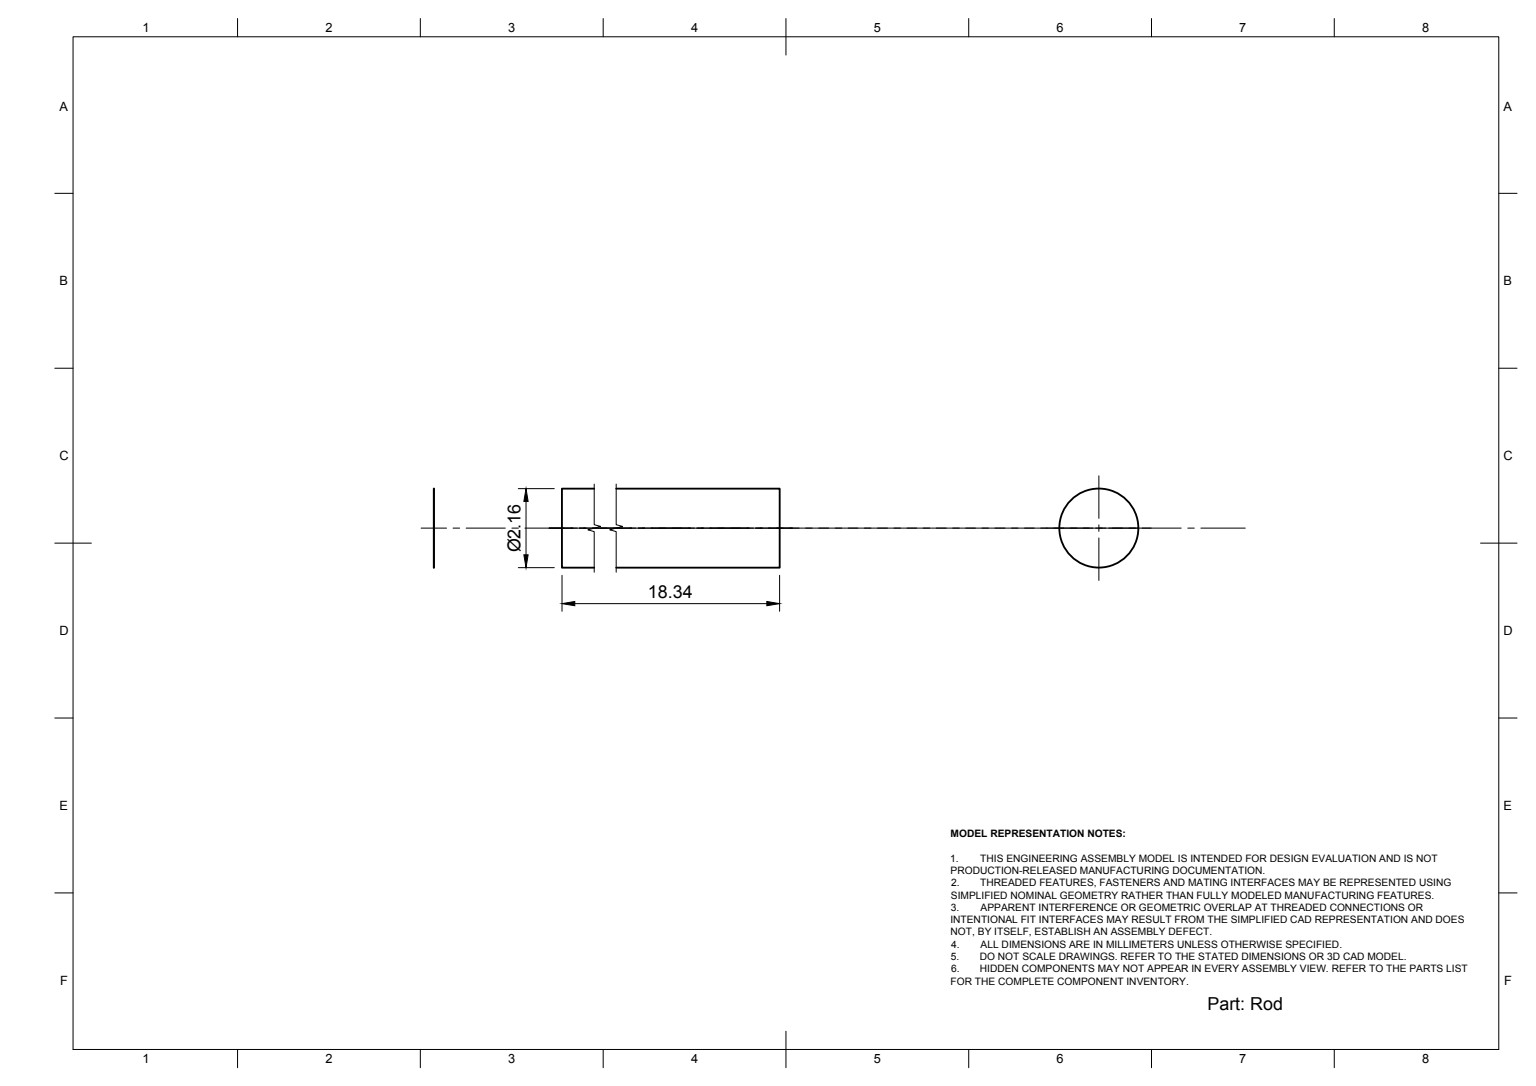
ISO-10303-21;
HEADER;
/* Generated by software containing ST-Developer
 * from STEP Tools, Inc. (www.steptools.com) 
 */

FILE_DESCRIPTION(
/* description */ (''),
/* implementation_level */ '2;1');

FILE_NAME(
/* name */ 'Rod.step',
/* time_stamp */ '2026-10-04T22:13:49-07:00',
/* author */ (''),
/* organization */ (''),
/* preprocessor_version */ 'ST-DEVELOPER v20.2',
/* originating_system */ 'Autodesk Translation Framework v15.15.0.0',
/* authorisation */ '');

FILE_SCHEMA (('AUTOMOTIVE_DESIGN { 1 0 10303 214 3 1 1 }'));
ENDSEC;

DATA;
#10=MECHANICAL_DESIGN_GEOMETRIC_PRESENTATION_REPRESENTATION('',(#365,#366),#40734);
#349=SHAPE_REPRESENTATION_RELATIONSHIP('SRR','None',#40770,#357);
#357=ADVANCED_BREP_SHAPE_REPRESENTATION('',(#374,#375),#40730);
#365=STYLED_ITEM('',(#40816),#374);
#366=STYLED_ITEM('',(#40816),#375);
#374=MANIFOLD_SOLID_BREP('Body1',#3170);
#375=MANIFOLD_SOLID_BREP('Body2',#3171);
#411=PLANE('',#3341);
#412=PLANE('',#3345);
#413=PLANE('',#3346);
#414=PLANE('',#3350);
#467=FACE_OUTER_BOUND('',#635,.T.);
#468=FACE_OUTER_BOUND('',#636,.T.);
#469=FACE_OUTER_BOUND('',#637,.T.);
#470=FACE_OUTER_BOUND('',#638,.T.);
#471=FACE_OUTER_BOUND('',#639,.T.);
#472=FACE_OUTER_BOUND('',#640,.T.);
#635=EDGE_LOOP('',(#2116));
#636=EDGE_LOOP('',(#2117,#2118,#2119,#2120));
#637=EDGE_LOOP('',(#2121));
#638=EDGE_LOOP('',(#2122));
#639=EDGE_LOOP('',(#2123,#2124,#2125,#2126));
#640=EDGE_LOOP('',(#2127));
#789=LINE('',#6473,#931);
#790=LINE('',#6481,#932);
#931=VECTOR('',#3674,1.08063175605657);
#932=VECTOR('',#3685,1.08063175605657);
#1074=CIRCLE('',#3342,1.08063175605657);
#1075=CIRCLE('',#3344,1.08063175605657);
#1076=CIRCLE('',#3347,1.08063175605657);
#1077=CIRCLE('',#3349,1.08063175605657);
#1159=VERTEX_POINT('',#6469);
#1160=VERTEX_POINT('',#6472);
#1161=VERTEX_POINT('',#6477);
#1162=VERTEX_POINT('',#6480);
#1534=EDGE_CURVE('',#1159,#1159,#1074,.T.);
#1535=EDGE_CURVE('',#1159,#1160,#789,.T.);
#1536=EDGE_CURVE('',#1160,#1160,#1075,.T.);
#1537=EDGE_CURVE('',#1161,#1161,#1076,.T.);
#1538=EDGE_CURVE('',#1161,#1162,#790,.T.);
#1539=EDGE_CURVE('',#1162,#1162,#1077,.T.);
#2116=ORIENTED_EDGE('',*,*,#1534,.F.);
#2117=ORIENTED_EDGE('',*,*,#1534,.T.);
#2118=ORIENTED_EDGE('',*,*,#1535,.T.);
#2119=ORIENTED_EDGE('',*,*,#1536,.T.);
#2120=ORIENTED_EDGE('',*,*,#1535,.F.);
#2121=ORIENTED_EDGE('',*,*,#1536,.F.);
#2122=ORIENTED_EDGE('',*,*,#1537,.T.);
#2123=ORIENTED_EDGE('',*,*,#1537,.F.);
#2124=ORIENTED_EDGE('',*,*,#1538,.T.);
#2125=ORIENTED_EDGE('',*,*,#1539,.T.);
#2126=ORIENTED_EDGE('',*,*,#1538,.F.);
#2127=ORIENTED_EDGE('',*,*,#1539,.F.);
#2908=CYLINDRICAL_SURFACE('',#3343,1.08063175605657);
#2909=CYLINDRICAL_SURFACE('',#3348,1.08063175605657);
#3046=ADVANCED_FACE('',(#467),#411,.F.);
#3047=ADVANCED_FACE('',(#468),#2908,.T.);
#3048=ADVANCED_FACE('',(#469),#412,.T.);
#3049=ADVANCED_FACE('',(#470),#413,.T.);
#3050=ADVANCED_FACE('',(#471),#2909,.T.);
#3051=ADVANCED_FACE('',(#472),#414,.T.);
#3170=CLOSED_SHELL('',(#3046,#3047,#3048));
#3171=CLOSED_SHELL('',(#3049,#3050,#3051));
#3340=AXIS2_PLACEMENT_3D('',#6467,#3666,#3667);
#3341=AXIS2_PLACEMENT_3D('',#6468,#3668,#3669);
#3342=AXIS2_PLACEMENT_3D('',#6470,#3670,#3671);
#3343=AXIS2_PLACEMENT_3D('',#6471,#3672,#3673);
#3344=AXIS2_PLACEMENT_3D('',#6474,#3675,#3676);
#3345=AXIS2_PLACEMENT_3D('',#6475,#3677,#3678);
#3346=AXIS2_PLACEMENT_3D('',#6476,#3679,#3680);
#3347=AXIS2_PLACEMENT_3D('',#6478,#3681,#3682);
#3348=AXIS2_PLACEMENT_3D('',#6479,#3683,#3684);
#3349=AXIS2_PLACEMENT_3D('',#6482,#3686,#3687);
#3350=AXIS2_PLACEMENT_3D('',#6483,#3688,#3689);
#3666=DIRECTION('axis',(0.,0.,1.));
#3667=DIRECTION('refdir',(1.,0.,0.));
#3668=DIRECTION('center_axis',(-1.,0.,0.));
#3669=DIRECTION('ref_axis',(0.,-1.,0.));
#3670=DIRECTION('center_axis',(-1.,0.,0.));
#3671=DIRECTION('ref_axis',(0.,0.,-1.));
#3672=DIRECTION('center_axis',(1.,0.,0.));
#3673=DIRECTION('ref_axis',(0.,0.,-1.));
#3674=DIRECTION('',(-1.,0.,0.));
#3675=DIRECTION('center_axis',(1.,0.,0.));
#3676=DIRECTION('ref_axis',(0.,0.,-1.));
#3677=DIRECTION('center_axis',(-1.,0.,0.));
#3678=DIRECTION('ref_axis',(0.,0.,1.));
#3679=DIRECTION('center_axis',(1.,0.,0.));
#3680=DIRECTION('ref_axis',(0.,0.,-1.));
#3681=DIRECTION('center_axis',(1.,0.,0.));
#3682=DIRECTION('ref_axis',(0.,0.,-1.));
#3683=DIRECTION('center_axis',(1.,0.,0.));
#3684=DIRECTION('ref_axis',(0.,0.,-1.));
#3685=DIRECTION('',(-1.,0.,0.));
#3686=DIRECTION('center_axis',(1.,0.,0.));
#3687=DIRECTION('ref_axis',(0.,0.,-1.));
#3688=DIRECTION('center_axis',(-1.,0.,0.));
#3689=DIRECTION('ref_axis',(0.,-1.,0.));
#6467=CARTESIAN_POINT('',(0.,0.,0.));
#6468=CARTESIAN_POINT('Origin',(85.6487002358236,0.,-8.18789480661053E-15));
#6469=CARTESIAN_POINT('',(85.6487002358236,-1.32339222111166E-16,1.08063175605657));
#6470=CARTESIAN_POINT('Origin',(85.6487002358236,0.,0.));
#6471=CARTESIAN_POINT('Origin',(78.2297384009075,0.,0.));
#6472=CARTESIAN_POINT('',(67.3063659679149,-1.32339222111166E-16,1.08063175605657));
#6473=CARTESIAN_POINT('',(78.2297384009075,-1.32339222111166E-16,1.08063175605657));
#6474=CARTESIAN_POINT('Origin',(67.3063659679149,0.,0.));
#6475=CARTESIAN_POINT('Origin',(67.3063659679149,0.,-1.08063175605657));
#6476=CARTESIAN_POINT('Origin',(89.1531108339,0.,0.));
#6477=CARTESIAN_POINT('',(89.1531108339,-1.32339222111166E-16,1.08063175605657));
#6478=CARTESIAN_POINT('Origin',(89.1531108339,0.,0.));
#6479=CARTESIAN_POINT('Origin',(78.2297384009075,0.,0.));
#6480=CARTESIAN_POINT('',(89.1487002358236,-1.32339222111166E-16,1.08063175605657));
#6481=CARTESIAN_POINT('',(78.2297384009075,-1.32339222111166E-16,1.08063175605657));
#6482=CARTESIAN_POINT('Origin',(89.1487002358236,0.,0.));
#6483=CARTESIAN_POINT('Origin',(89.1487002358236,0.,-8.18789480661053E-15));
#40720=UNCERTAINTY_MEASURE_WITH_UNIT(LENGTH_MEASURE(0.01),#40735,
'DISTANCE_ACCURACY_VALUE',
'Maximum model space distance between geometric entities at asserted c
onnectivities');
#40724=UNCERTAINTY_MEASURE_WITH_UNIT(LENGTH_MEASURE(0.01),#40735,
'DISTANCE_ACCURACY_VALUE',
'Maximum model space distance between geometric entities at asserted c
onnectivities');
#40730=(
GEOMETRIC_REPRESENTATION_CONTEXT(3)
GLOBAL_UNCERTAINTY_ASSIGNED_CONTEXT((#40720))
GLOBAL_UNIT_ASSIGNED_CONTEXT((#40735,#40737,#40738))
REPRESENTATION_CONTEXT('','3D')
);
#40734=(
GEOMETRIC_REPRESENTATION_CONTEXT(3)
GLOBAL_UNCERTAINTY_ASSIGNED_CONTEXT((#40724))
GLOBAL_UNIT_ASSIGNED_CONTEXT((#40735,#40737,#40738))
REPRESENTATION_CONTEXT('','3D')
);
#40735=(
LENGTH_UNIT()
NAMED_UNIT(*)
SI_UNIT(.MILLI.,.METRE.)
);
#40737=(
NAMED_UNIT(*)
PLANE_ANGLE_UNIT()
SI_UNIT($,.RADIAN.)
);
#40738=(
NAMED_UNIT(*)
SI_UNIT($,.STERADIAN.)
SOLID_ANGLE_UNIT()
);
#40744=SHAPE_DEFINITION_REPRESENTATION(#40753,#40770);
#40753=PRODUCT_DEFINITION_SHAPE('',$,#40780);
#40770=SHAPE_REPRESENTATION('',(#3340),#40730);
#40774=PRODUCT_DEFINITION_CONTEXT('part definition',#40803,'design');
#40780=PRODUCT_DEFINITION('Rod','Rod',#40789,#40774);
#40789=PRODUCT_DEFINITION_FORMATION('',$,#40810);
#40803=APPLICATION_CONTEXT(
'Core Data for Automotive Mechanical Design Process');
#40804=PRODUCT_CONTEXT('part definition',#40803,'mechanical');
#40810=PRODUCT('Rod','Rod',$,(#40804));
#40816=PRESENTATION_STYLE_ASSIGNMENT((#40819));
#40819=SURFACE_STYLE_USAGE(.BOTH.,#40822);
#40822=SURFACE_SIDE_STYLE('',(#40825));
#40825=SURFACE_STYLE_FILL_AREA(#40828);
#40828=FILL_AREA_STYLE('Opaque(67,67,67)',(#40831));
#40831=FILL_AREA_STYLE_COLOUR('Opaque(67,67,67)',#40834);
#40834=COLOUR_RGB('Opaque(67,67,67)', 0.66274510, 0.83137255, 0.94901961);
ENDSEC;
END-ISO-10303-21;
